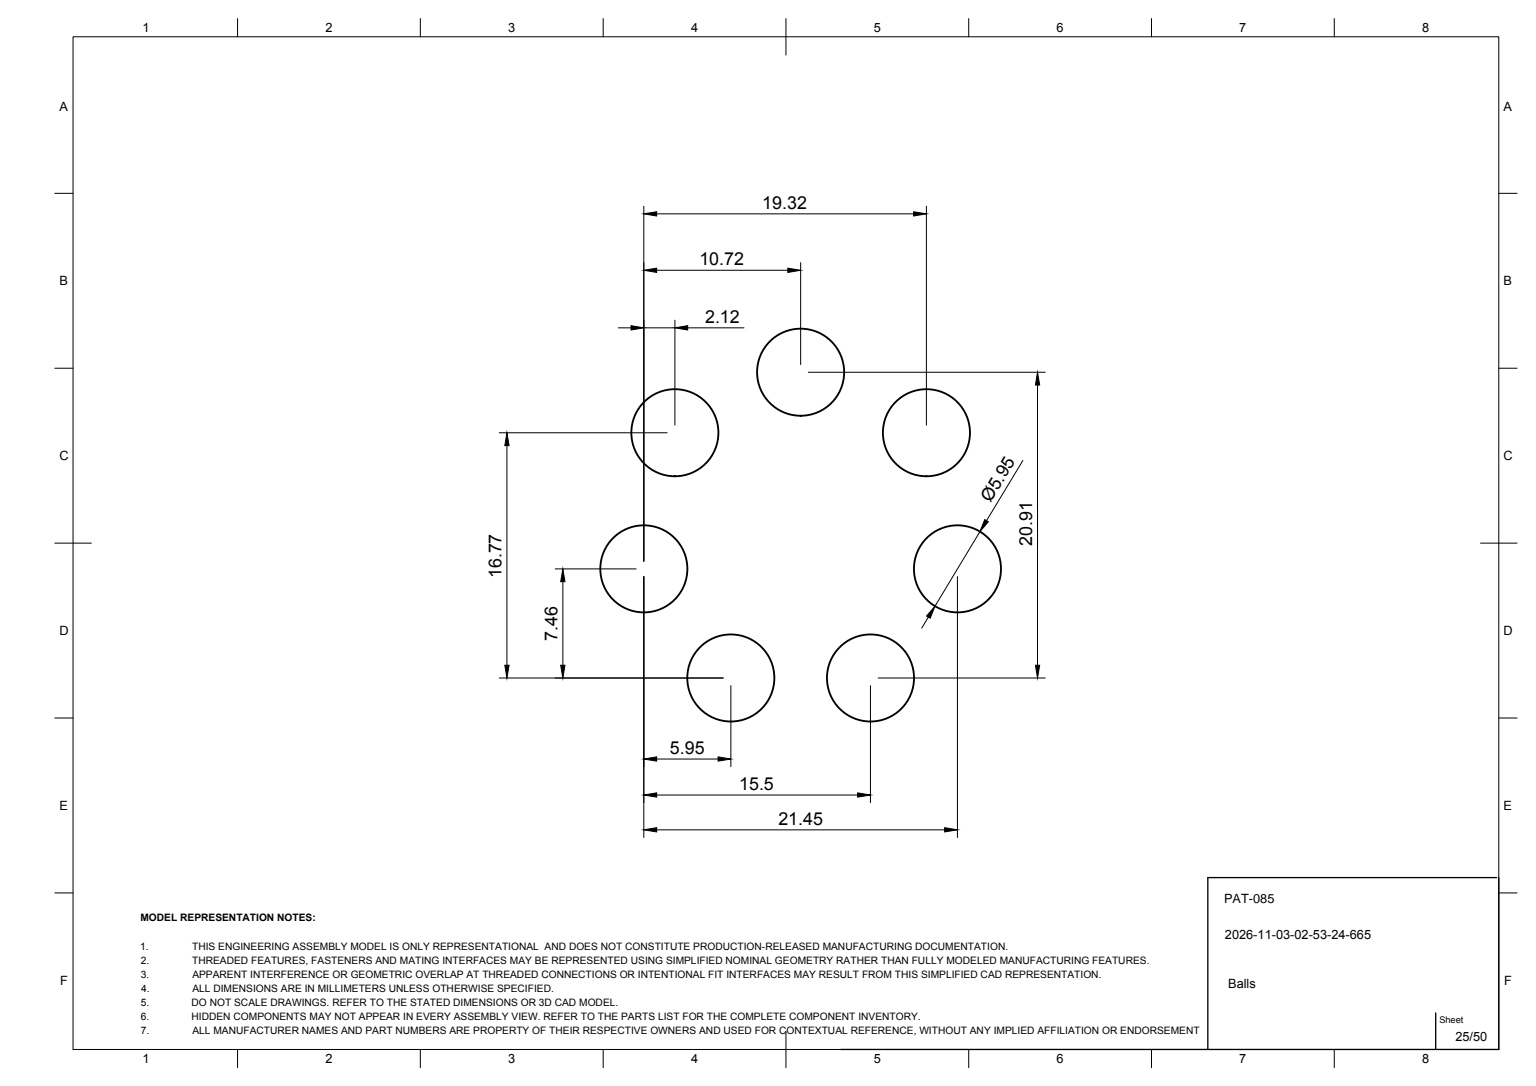
ISO-10303-21;
HEADER;
/* Generated by software containing ST-Developer
 * from STEP Tools, Inc. (www.steptools.com) 
 */

FILE_DESCRIPTION(
/* description */ ('Rack and pinion manual slide'),
/* implementation_level */ '2;1');

FILE_NAME(
/* name */ 'Balls.step',
/* time_stamp */ '2026-10-28T03:22:49-07:00',
/* author */ (''),
/* organization */ (''),
/* preprocessor_version */ 'ST-DEVELOPER v20.2',
/* originating_system */ 'Autodesk Translation Framework v15.17.0.0',
/* authorisation */ '');

FILE_SCHEMA (('AUTOMOTIVE_DESIGN { 1 0 10303 214 3 1 1 }'));
ENDSEC;

DATA;
#10=MECHANICAL_DESIGN_GEOMETRIC_PRESENTATION_REPRESENTATION('',(#753,#754,#755,#756,#757,#758,#759),#34851);
#589=SPHERICAL_SURFACE('',#14820,0.29765);
#590=SPHERICAL_SURFACE('',#14822,0.29765);
#591=SPHERICAL_SURFACE('',#14824,0.29765);
#592=SPHERICAL_SURFACE('',#14826,0.29765);
#593=SPHERICAL_SURFACE('',#14828,0.29765);
#594=SPHERICAL_SURFACE('',#14830,0.29765);
#595=SPHERICAL_SURFACE('',#14832,0.29765);
#661=SHAPE_REPRESENTATION_RELATIONSHIP('SRR','None',#35097,#707);
#707=ADVANCED_BREP_SHAPE_REPRESENTATION('',(#805,#806,#807,#808,#809,#810,
#811),#34822);
#753=STYLED_ITEM('',(#35411),#805);
#754=STYLED_ITEM('',(#35411),#806);
#755=STYLED_ITEM('',(#35411),#807);
#756=STYLED_ITEM('',(#35411),#808);
#757=STYLED_ITEM('',(#35411),#809);
#758=STYLED_ITEM('',(#35411),#810);
#759=STYLED_ITEM('',(#35411),#811);
#805=MANIFOLD_SOLID_BREP('Body1',#13774);
#806=MANIFOLD_SOLID_BREP('Body2',#13775);
#807=MANIFOLD_SOLID_BREP('Body3',#13776);
#808=MANIFOLD_SOLID_BREP('Body4',#13777);
#809=MANIFOLD_SOLID_BREP('Body5',#13778);
#810=MANIFOLD_SOLID_BREP('Body6',#13779);
#811=MANIFOLD_SOLID_BREP('Body7',#13780);
#1814=FACE_OUTER_BOUND('',#2699,.T.);
#1815=FACE_OUTER_BOUND('',#2700,.T.);
#1816=FACE_OUTER_BOUND('',#2701,.T.);
#1817=FACE_OUTER_BOUND('',#2702,.T.);
#1818=FACE_OUTER_BOUND('',#2703,.T.);
#1819=FACE_OUTER_BOUND('',#2704,.T.);
#1820=FACE_OUTER_BOUND('',#2705,.T.);
#2699=EDGE_LOOP('',(#10554,#10555));
#2700=EDGE_LOOP('',(#10556,#10557));
#2701=EDGE_LOOP('',(#10558,#10559));
#2702=EDGE_LOOP('',(#10560,#10561));
#2703=EDGE_LOOP('',(#10562,#10563));
#2704=EDGE_LOOP('',(#10564,#10565));
#2705=EDGE_LOOP('',(#10566,#10567));
#6003=CIRCLE('',#14821,0.29765);
#6004=CIRCLE('',#14823,0.29765);
#6005=CIRCLE('',#14825,0.29765);
#6006=CIRCLE('',#14827,0.29765);
#6007=CIRCLE('',#14829,0.29765);
#6008=CIRCLE('',#14831,0.29765);
#6009=CIRCLE('',#14833,0.29765);
#6661=VERTEX_POINT('',#20859);
#6662=VERTEX_POINT('',#20860);
#6663=VERTEX_POINT('',#20863);
#6664=VERTEX_POINT('',#20864);
#6665=VERTEX_POINT('',#20867);
#6666=VERTEX_POINT('',#20868);
#6667=VERTEX_POINT('',#20871);
#6668=VERTEX_POINT('',#20872);
#6669=VERTEX_POINT('',#20875);
#6670=VERTEX_POINT('',#20876);
#6671=VERTEX_POINT('',#20879);
#6672=VERTEX_POINT('',#20880);
#6673=VERTEX_POINT('',#20883);
#6674=VERTEX_POINT('',#20884);
#8089=EDGE_CURVE('',#6661,#6662,#6003,.T.);
#8090=EDGE_CURVE('',#6663,#6664,#6004,.T.);
#8091=EDGE_CURVE('',#6665,#6666,#6005,.T.);
#8092=EDGE_CURVE('',#6667,#6668,#6006,.T.);
#8093=EDGE_CURVE('',#6669,#6670,#6007,.T.);
#8094=EDGE_CURVE('',#6671,#6672,#6008,.T.);
#8095=EDGE_CURVE('',#6673,#6674,#6009,.T.);
#10554=ORIENTED_EDGE('',*,*,#8089,.T.);
#10555=ORIENTED_EDGE('',*,*,#8089,.F.);
#10556=ORIENTED_EDGE('',*,*,#8090,.T.);
#10557=ORIENTED_EDGE('',*,*,#8090,.F.);
#10558=ORIENTED_EDGE('',*,*,#8091,.T.);
#10559=ORIENTED_EDGE('',*,*,#8091,.F.);
#10560=ORIENTED_EDGE('',*,*,#8092,.T.);
#10561=ORIENTED_EDGE('',*,*,#8092,.F.);
#10562=ORIENTED_EDGE('',*,*,#8093,.T.);
#10563=ORIENTED_EDGE('',*,*,#8093,.F.);
#10564=ORIENTED_EDGE('',*,*,#8094,.T.);
#10565=ORIENTED_EDGE('',*,*,#8094,.F.);
#10566=ORIENTED_EDGE('',*,*,#8095,.T.);
#10567=ORIENTED_EDGE('',*,*,#8095,.F.);
#13292=ADVANCED_FACE('',(#1814),#589,.T.);
#13293=ADVANCED_FACE('',(#1815),#590,.T.);
#13294=ADVANCED_FACE('',(#1816),#591,.T.);
#13295=ADVANCED_FACE('',(#1817),#592,.T.);
#13296=ADVANCED_FACE('',(#1818),#593,.T.);
#13297=ADVANCED_FACE('',(#1819),#594,.T.);
#13298=ADVANCED_FACE('',(#1820),#595,.T.);
#13774=CLOSED_SHELL('',(#13292));
#13775=CLOSED_SHELL('',(#13293));
#13776=CLOSED_SHELL('',(#13294));
#13777=CLOSED_SHELL('',(#13295));
#13778=CLOSED_SHELL('',(#13296));
#13779=CLOSED_SHELL('',(#13297));
#13780=CLOSED_SHELL('',(#13298));
#14819=AXIS2_PLACEMENT_3D('',#20857,#17065,#17066);
#14820=AXIS2_PLACEMENT_3D('',#20858,#17067,#17068);
#14821=AXIS2_PLACEMENT_3D('',#20861,#17069,#17070);
#14822=AXIS2_PLACEMENT_3D('',#20862,#17071,#17072);
#14823=AXIS2_PLACEMENT_3D('',#20865,#17073,#17074);
#14824=AXIS2_PLACEMENT_3D('',#20866,#17075,#17076);
#14825=AXIS2_PLACEMENT_3D('',#20869,#17077,#17078);
#14826=AXIS2_PLACEMENT_3D('',#20870,#17079,#17080);
#14827=AXIS2_PLACEMENT_3D('',#20873,#17081,#17082);
#14828=AXIS2_PLACEMENT_3D('',#20874,#17083,#17084);
#14829=AXIS2_PLACEMENT_3D('',#20877,#17085,#17086);
#14830=AXIS2_PLACEMENT_3D('',#20878,#17087,#17088);
#14831=AXIS2_PLACEMENT_3D('',#20881,#17089,#17090);
#14832=AXIS2_PLACEMENT_3D('',#20882,#17091,#17092);
#14833=AXIS2_PLACEMENT_3D('',#20885,#17093,#17094);
#17065=DIRECTION('axis',(0.,0.,1.));
#17066=DIRECTION('refdir',(1.,0.,0.));
#17067=DIRECTION('center_axis',(0.,0.,1.));
#17068=DIRECTION('ref_axis',(1.,0.,0.));
#17069=DIRECTION('center_axis',(1.22464679914735E-16,-1.,0.));
#17070=DIRECTION('ref_axis',(-1.,-1.22464679914735E-16,0.));
#17071=DIRECTION('center_axis',(0.78183148246803,0.,0.623489801858733));
#17072=DIRECTION('ref_axis',(0.623489801858734,0.,-0.78183148246803));
#17073=DIRECTION('center_axis',(7.63554790147315E-17,-1.,-9.57467422477103E-17));
#17074=DIRECTION('ref_axis',(-0.623489801858734,-1.22464679914735E-16,0.78183148246803));
#17075=DIRECTION('center_axis',(0.974927912181824,0.,-0.222520933956314));
#17076=DIRECTION('ref_axis',(-0.222520933956314,0.,-0.974927912181824));
#17077=DIRECTION('center_axis',(-2.7250954951288E-17,-1.,-1.19394234705288E-16));
#17078=DIRECTION('ref_axis',(0.222520933956314,-1.22464679914735E-16,0.974927912181824));
#17079=DIRECTION('center_axis',(0.433883739117558,0.,-0.900968867902419));
#17080=DIRECTION('ref_axis',(-0.900968867902419,0.,-0.433883739117558));
#17081=DIRECTION('center_axis',(-1.10336864020811E-16,-1.,-5.31354332312403E-17));
#17082=DIRECTION('ref_axis',(0.900968867902419,-1.22464679914735E-16,0.433883739117558));
#17083=DIRECTION('center_axis',(-0.433883739117558,0.,-0.900968867902419));
#17084=DIRECTION('ref_axis',(-0.900968867902419,0.,0.433883739117558));
#17085=DIRECTION('center_axis',(-1.10336864020811E-16,-1.,5.31354332312403E-17));
#17086=DIRECTION('ref_axis',(0.900968867902419,-1.22464679914735E-16,-0.433883739117558));
#17087=DIRECTION('center_axis',(-0.974927912181824,0.,-0.222520933956314));
#17088=DIRECTION('ref_axis',(-0.222520933956315,0.,0.974927912181824));
#17089=DIRECTION('center_axis',(-2.7250954951288E-17,-1.,1.19394234705288E-16));
#17090=DIRECTION('ref_axis',(0.222520933956315,-1.22464679914735E-16,-0.974927912181824));
#17091=DIRECTION('center_axis',(-0.78183148246803,0.,0.623489801858734));
#17092=DIRECTION('ref_axis',(0.623489801858733,0.,0.78183148246803));
#17093=DIRECTION('center_axis',(7.63554790147315E-17,-1.,9.57467422477103E-17));
#17094=DIRECTION('ref_axis',(-0.623489801858733,-1.22464679914735E-16,-0.78183148246803));
#20857=CARTESIAN_POINT('',(0.,0.,0.));
#20858=CARTESIAN_POINT('Origin',(1.1,0.,0.));
#20859=CARTESIAN_POINT('',(1.1,-2.23201749654651E-33,0.29765));
#20860=CARTESIAN_POINT('',(1.1,-2.23201749654651E-33,-0.29765));
#20861=CARTESIAN_POINT('Origin',(1.1,0.,0.));
#20862=CARTESIAN_POINT('Origin',(0.685838782044607,0.,-0.860014630714833));
#20863=CARTESIAN_POINT('',(0.918550922801216,-5.31350540756609E-33,-0.674432891191581));
#20864=CARTESIAN_POINT('',(0.453126641287998,8.49470414473068E-34,-1.04559637023808));
#20865=CARTESIAN_POINT('Origin',(0.685838782044607,0.,-0.860014630714833));
#20866=CARTESIAN_POINT('Origin',(-0.244773027351946,0.,-1.07242070340001));
#20867=CARTESIAN_POINT('',(0.0454142657089739,-2.23201749654651E-33,-1.1386540593921));
#20868=CARTESIAN_POINT('',(-0.534960320412865,-2.23201749654651E-33,-1.00618734740791));
#20869=CARTESIAN_POINT('Origin',(-0.244773027351946,0.,-1.07242070340001));
#20870=CARTESIAN_POINT('Origin',(-0.991065754692661,0.,-0.477272113029314));
#20871=CARTESIAN_POINT('',(-0.86192025974432,8.49470414473067E-34,-0.745445496560469));
#20872=CARTESIAN_POINT('',(-1.120211249641,-5.31350540756609E-33,-0.209098729498159));
#20873=CARTESIAN_POINT('Origin',(-0.991065754692661,0.,-0.477272113029314));
#20874=CARTESIAN_POINT('Origin',(-0.991065754692661,0.,0.477272113029314));
#20875=CARTESIAN_POINT('',(-1.120211249641,-2.23201749654651E-33,0.209098729498159));
#20876=CARTESIAN_POINT('',(-0.86192025974432,-2.23201749654651E-33,0.745445496560469));
#20877=CARTESIAN_POINT('Origin',(-0.991065754692661,0.,0.477272113029314));
#20878=CARTESIAN_POINT('Origin',(-0.244773027351946,0.,1.07242070340001));
#20879=CARTESIAN_POINT('',(-0.534960320412866,-2.23201749654651E-33,1.00618734740791));
#20880=CARTESIAN_POINT('',(0.0454142657089737,-2.23201749654651E-33,1.1386540593921));
#20881=CARTESIAN_POINT('Origin',(-0.244773027351946,0.,1.07242070340001));
#20882=CARTESIAN_POINT('Origin',(0.685838782044607,0.,0.860014630714833));
#20883=CARTESIAN_POINT('',(0.453126641287998,-2.23201749654651E-33,1.04559637023808));
#20884=CARTESIAN_POINT('',(0.918550922801216,-2.23201749654651E-33,0.674432891191581));
#20885=CARTESIAN_POINT('Origin',(0.685838782044607,0.,0.860014630714833));
#34768=UNCERTAINTY_MEASURE_WITH_UNIT(LENGTH_MEASURE(0.001),#34852,
'DISTANCE_ACCURACY_VALUE',
'Maximum model space distance between geometric entities at asserted c
onnectivities');
#34797=UNCERTAINTY_MEASURE_WITH_UNIT(LENGTH_MEASURE(0.001),#34852,
'DISTANCE_ACCURACY_VALUE',
'Maximum model space distance between geometric entities at asserted c
onnectivities');
#34822=(
GEOMETRIC_REPRESENTATION_CONTEXT(3)
GLOBAL_UNCERTAINTY_ASSIGNED_CONTEXT((#34768))
GLOBAL_UNIT_ASSIGNED_CONTEXT((#34852,#34854,#34855))
REPRESENTATION_CONTEXT('','3D')
);
#34851=(
GEOMETRIC_REPRESENTATION_CONTEXT(3)
GLOBAL_UNCERTAINTY_ASSIGNED_CONTEXT((#34797))
GLOBAL_UNIT_ASSIGNED_CONTEXT((#34852,#34854,#34855))
REPRESENTATION_CONTEXT('','3D')
);
#34852=(
LENGTH_UNIT()
NAMED_UNIT(*)
SI_UNIT(.CENTI.,.METRE.)
);
#34854=(
NAMED_UNIT(*)
PLANE_ANGLE_UNIT()
SI_UNIT($,.RADIAN.)
);
#34855=(
NAMED_UNIT(*)
SI_UNIT($,.STERADIAN.)
SOLID_ANGLE_UNIT()
);
#34880=SHAPE_DEFINITION_REPRESENTATION(#34933,#35097);
#34933=PRODUCT_DEFINITION_SHAPE('',$,#35151);
#35097=SHAPE_REPRESENTATION('',(#14819),#34822);
#35126=PRODUCT_DEFINITION_CONTEXT('part definition',#35287,'design');
#35151=PRODUCT_DEFINITION('Balls','Balls',#35204,#35126);
#35204=PRODUCT_DEFINITION_FORMATION('',$,#35313);
#35287=APPLICATION_CONTEXT(
'Core Data for Automotive Mechanical Design Process');
#35288=PRODUCT_CONTEXT('part definition',#35287,'mechanical');
#35313=PRODUCT('Balls','Balls','Balls',(#35288));
#35405=COLOUR_RGB('Grey',0.48,0.52,0.57);
#35406=FILL_AREA_STYLE_COLOUR('',#35405);
#35407=FILL_AREA_STYLE('',(#35406));
#35408=SURFACE_STYLE_FILL_AREA(#35407);
#35409=SURFACE_SIDE_STYLE('',(#35408));
#35410=SURFACE_STYLE_USAGE(.BOTH.,#35409);
#35411=PRESENTATION_STYLE_ASSIGNMENT((#35410));
ENDSEC;
END-ISO-10303-21;
